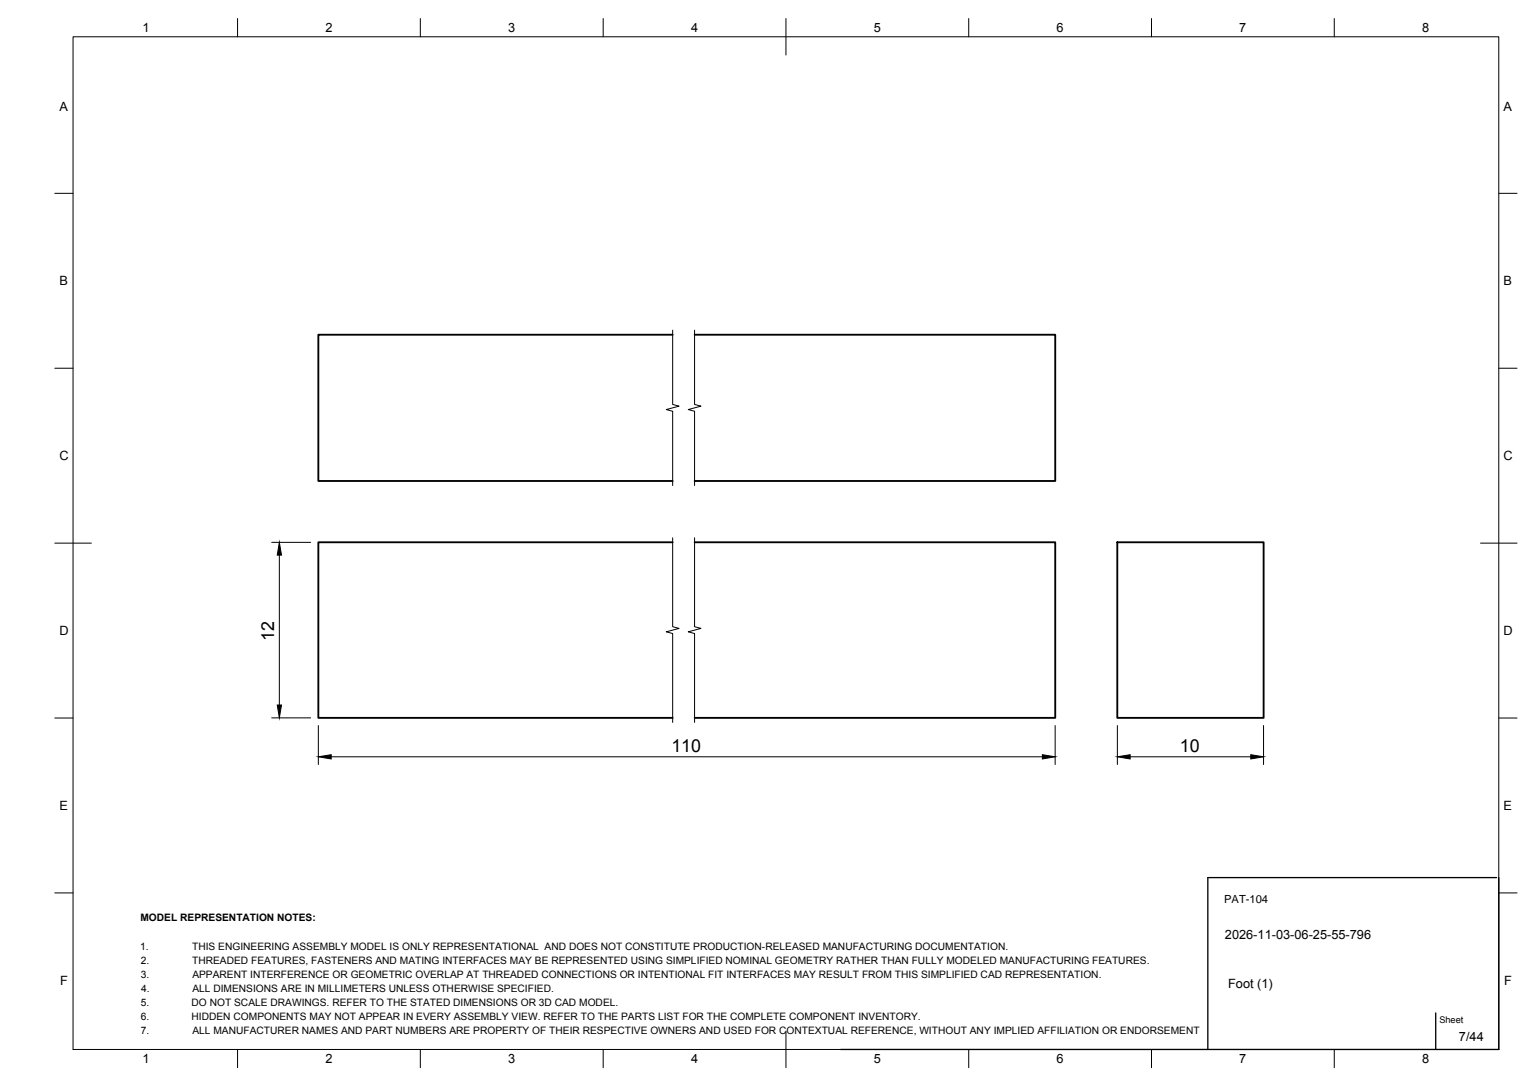
ISO-10303-21;
HEADER;
/* Generated by software containing ST-Developer
 * from STEP Tools, Inc. (www.steptools.com) 
 */

FILE_DESCRIPTION(
/* description */ ('Timing belt drive module 2 mm Pitch Timing 20T-40T'),

/* implementation_level */ '2;1');

FILE_NAME(
/* name */ 'Foot (1).step',
/* time_stamp */ '2026-10-28T03:25:12-07:00',
/* author */ (''),
/* organization */ (''),
/* preprocessor_version */ 'ST-DEVELOPER v20.2',
/* originating_system */ 'Autodesk Translation Framework v15.17.0.0',
/* authorisation */ '');

FILE_SCHEMA (('AUTOMOTIVE_DESIGN { 1 0 10303 214 3 1 1 }'));
ENDSEC;

DATA;
#10=MECHANICAL_DESIGN_GEOMETRIC_PRESENTATION_REPRESENTATION('',(#526),#17830);
#440=SHAPE_REPRESENTATION_RELATIONSHIP('SRR','None',#18010,#483);
#483=ADVANCED_BREP_SHAPE_REPRESENTATION('',(#584),#17785);
#526=STYLED_ITEM('',(#18331),#584);
#584=MANIFOLD_SOLID_BREP('Body1',#8983);
#797=PLANE('',#9585);
#798=PLANE('',#9586);
#799=PLANE('',#9587);
#800=PLANE('',#9588);
#801=PLANE('',#9589);
#802=PLANE('',#9590);
#998=FACE_OUTER_BOUND('',#1529,.T.);
#999=FACE_OUTER_BOUND('',#1530,.T.);
#1000=FACE_OUTER_BOUND('',#1531,.T.);
#1001=FACE_OUTER_BOUND('',#1532,.T.);
#1002=FACE_OUTER_BOUND('',#1533,.T.);
#1003=FACE_OUTER_BOUND('',#1534,.T.);
#1529=EDGE_LOOP('',(#5953,#5954,#5955,#5956));
#1530=EDGE_LOOP('',(#5957,#5958,#5959,#5960));
#1531=EDGE_LOOP('',(#5961,#5962,#5963,#5964));
#1532=EDGE_LOOP('',(#5965,#5966,#5967,#5968));
#1533=EDGE_LOOP('',(#5969,#5970,#5971,#5972));
#1534=EDGE_LOOP('',(#5973,#5974,#5975,#5976));
#2852=LINE('',#14067,#3330);
#2853=LINE('',#14069,#3331);
#2854=LINE('',#14071,#3332);
#2855=LINE('',#14072,#3333);
#2856=LINE('',#14075,#3334);
#2857=LINE('',#14077,#3335);
#2858=LINE('',#14078,#3336);
#2859=LINE('',#14081,#3337);
#2860=LINE('',#14083,#3338);
#2861=LINE('',#14084,#3339);
#2862=LINE('',#14086,#3340);
#2863=LINE('',#14087,#3341);
#3330=VECTOR('',#11011,1.);
#3331=VECTOR('',#11012,1.);
#3332=VECTOR('',#11013,1.);
#3333=VECTOR('',#11014,1.);
#3334=VECTOR('',#11017,1.);
#3335=VECTOR('',#11018,1.);
#3336=VECTOR('',#11019,1.);
#3337=VECTOR('',#11022,1.);
#3338=VECTOR('',#11023,1.);
#3339=VECTOR('',#11024,1.);
#3340=VECTOR('',#11027,1.);
#3341=VECTOR('',#11028,1.);
#3806=VERTEX_POINT('',#14065);
#3807=VERTEX_POINT('',#14066);
#3808=VERTEX_POINT('',#14068);
#3809=VERTEX_POINT('',#14070);
#3810=VERTEX_POINT('',#14074);
#3811=VERTEX_POINT('',#14076);
#3812=VERTEX_POINT('',#14080);
#3813=VERTEX_POINT('',#14082);
#4659=EDGE_CURVE('',#3806,#3807,#2852,.T.);
#4660=EDGE_CURVE('',#3807,#3808,#2853,.T.);
#4661=EDGE_CURVE('',#3809,#3808,#2854,.T.);
#4662=EDGE_CURVE('',#3806,#3809,#2855,.T.);
#4663=EDGE_CURVE('',#3810,#3806,#2856,.T.);
#4664=EDGE_CURVE('',#3811,#3809,#2857,.T.);
#4665=EDGE_CURVE('',#3810,#3811,#2858,.T.);
#4666=EDGE_CURVE('',#3812,#3810,#2859,.T.);
#4667=EDGE_CURVE('',#3813,#3811,#2860,.T.);
#4668=EDGE_CURVE('',#3812,#3813,#2861,.T.);
#4669=EDGE_CURVE('',#3807,#3812,#2862,.T.);
#4670=EDGE_CURVE('',#3808,#3813,#2863,.T.);
#5953=ORIENTED_EDGE('',*,*,#4659,.T.);
#5954=ORIENTED_EDGE('',*,*,#4660,.T.);
#5955=ORIENTED_EDGE('',*,*,#4661,.F.);
#5956=ORIENTED_EDGE('',*,*,#4662,.F.);
#5957=ORIENTED_EDGE('',*,*,#4663,.T.);
#5958=ORIENTED_EDGE('',*,*,#4662,.T.);
#5959=ORIENTED_EDGE('',*,*,#4664,.F.);
#5960=ORIENTED_EDGE('',*,*,#4665,.F.);
#5961=ORIENTED_EDGE('',*,*,#4666,.T.);
#5962=ORIENTED_EDGE('',*,*,#4665,.T.);
#5963=ORIENTED_EDGE('',*,*,#4667,.F.);
#5964=ORIENTED_EDGE('',*,*,#4668,.F.);
#5965=ORIENTED_EDGE('',*,*,#4669,.T.);
#5966=ORIENTED_EDGE('',*,*,#4668,.T.);
#5967=ORIENTED_EDGE('',*,*,#4670,.F.);
#5968=ORIENTED_EDGE('',*,*,#4660,.F.);
#5969=ORIENTED_EDGE('',*,*,#4670,.T.);
#5970=ORIENTED_EDGE('',*,*,#4667,.T.);
#5971=ORIENTED_EDGE('',*,*,#4664,.T.);
#5972=ORIENTED_EDGE('',*,*,#4661,.T.);
#5973=ORIENTED_EDGE('',*,*,#4669,.F.);
#5974=ORIENTED_EDGE('',*,*,#4659,.F.);
#5975=ORIENTED_EDGE('',*,*,#4663,.F.);
#5976=ORIENTED_EDGE('',*,*,#4666,.F.);
#8496=ADVANCED_FACE('',(#998),#797,.T.);
#8497=ADVANCED_FACE('',(#999),#798,.T.);
#8498=ADVANCED_FACE('',(#1000),#799,.T.);
#8499=ADVANCED_FACE('',(#1001),#800,.T.);
#8500=ADVANCED_FACE('',(#1002),#801,.T.);
#8501=ADVANCED_FACE('',(#1003),#802,.F.);
#8983=CLOSED_SHELL('',(#8496,#8497,#8498,#8499,#8500,#8501));
#9584=AXIS2_PLACEMENT_3D('',#14063,#11007,#11008);
#9585=AXIS2_PLACEMENT_3D('',#14064,#11009,#11010);
#9586=AXIS2_PLACEMENT_3D('',#14073,#11015,#11016);
#9587=AXIS2_PLACEMENT_3D('',#14079,#11020,#11021);
#9588=AXIS2_PLACEMENT_3D('',#14085,#11025,#11026);
#9589=AXIS2_PLACEMENT_3D('',#14088,#11029,#11030);
#9590=AXIS2_PLACEMENT_3D('',#14089,#11031,#11032);
#11007=DIRECTION('axis',(0.,0.,1.));
#11008=DIRECTION('refdir',(1.,0.,0.));
#11009=DIRECTION('center_axis',(0.,1.,0.));
#11010=DIRECTION('ref_axis',(-1.,0.,0.));
#11011=DIRECTION('',(-1.,0.,0.));
#11012=DIRECTION('',(0.,0.,1.));
#11013=DIRECTION('',(-1.,0.,0.));
#11014=DIRECTION('',(0.,0.,1.));
#11015=DIRECTION('center_axis',(1.,0.,0.));
#11016=DIRECTION('ref_axis',(0.,1.,0.));
#11017=DIRECTION('',(0.,1.,0.));
#11018=DIRECTION('',(0.,1.,0.));
#11019=DIRECTION('',(0.,0.,1.));
#11020=DIRECTION('center_axis',(0.,-1.,0.));
#11021=DIRECTION('ref_axis',(1.,0.,0.));
#11022=DIRECTION('',(1.,0.,0.));
#11023=DIRECTION('',(1.,0.,0.));
#11024=DIRECTION('',(0.,0.,1.));
#11025=DIRECTION('center_axis',(-1.,0.,0.));
#11026=DIRECTION('ref_axis',(0.,-1.,0.));
#11027=DIRECTION('',(0.,-1.,0.));
#11028=DIRECTION('',(0.,-1.,0.));
#11029=DIRECTION('center_axis',(0.,0.,1.));
#11030=DIRECTION('ref_axis',(1.,0.,0.));
#11031=DIRECTION('center_axis',(0.,0.,1.));
#11032=DIRECTION('ref_axis',(1.,0.,0.));
#14063=CARTESIAN_POINT('',(0.,0.,0.));
#14064=CARTESIAN_POINT('Origin',(12.,4.5,-2.4));
#14065=CARTESIAN_POINT('',(12.,4.5,-2.4));
#14066=CARTESIAN_POINT('',(11.,4.5,-2.4));
#14067=CARTESIAN_POINT('',(12.,4.5,-2.4));
#14068=CARTESIAN_POINT('',(11.,4.5,-1.2));
#14069=CARTESIAN_POINT('',(11.,4.5,-2.4));
#14070=CARTESIAN_POINT('',(12.,4.5,-1.2));
#14071=CARTESIAN_POINT('',(12.,4.5,-1.2));
#14072=CARTESIAN_POINT('',(12.,4.5,-2.4));
#14073=CARTESIAN_POINT('Origin',(12.,-6.5,-2.4));
#14074=CARTESIAN_POINT('',(12.,-6.5,-2.4));
#14075=CARTESIAN_POINT('',(12.,-6.5,-2.4));
#14076=CARTESIAN_POINT('',(12.,-6.5,-1.2));
#14077=CARTESIAN_POINT('',(12.,-6.5,-1.2));
#14078=CARTESIAN_POINT('',(12.,-6.5,-2.4));
#14079=CARTESIAN_POINT('Origin',(11.,-6.5,-2.4));
#14080=CARTESIAN_POINT('',(11.,-6.5,-2.4));
#14081=CARTESIAN_POINT('',(11.,-6.5,-2.4));
#14082=CARTESIAN_POINT('',(11.,-6.5,-1.2));
#14083=CARTESIAN_POINT('',(11.,-6.5,-1.2));
#14084=CARTESIAN_POINT('',(11.,-6.5,-2.4));
#14085=CARTESIAN_POINT('Origin',(11.,4.5,-2.4));
#14086=CARTESIAN_POINT('',(11.,4.5,-2.4));
#14087=CARTESIAN_POINT('',(11.,4.5,-1.2));
#14088=CARTESIAN_POINT('Origin',(11.5,-1.,-1.2));
#14089=CARTESIAN_POINT('Origin',(11.5,-1.,-2.4));
#17735=UNCERTAINTY_MEASURE_WITH_UNIT(LENGTH_MEASURE(0.001),#17831,
'DISTANCE_ACCURACY_VALUE',
'Maximum model space distance between geometric entities at asserted c
onnectivities');
#17780=UNCERTAINTY_MEASURE_WITH_UNIT(LENGTH_MEASURE(0.001),#17831,
'DISTANCE_ACCURACY_VALUE',
'Maximum model space distance between geometric entities at asserted c
onnectivities');
#17785=(
GEOMETRIC_REPRESENTATION_CONTEXT(3)
GLOBAL_UNCERTAINTY_ASSIGNED_CONTEXT((#17735))
GLOBAL_UNIT_ASSIGNED_CONTEXT((#17831,#17833,#17834))
REPRESENTATION_CONTEXT('','3D')
);
#17830=(
GEOMETRIC_REPRESENTATION_CONTEXT(3)
GLOBAL_UNCERTAINTY_ASSIGNED_CONTEXT((#17780))
GLOBAL_UNIT_ASSIGNED_CONTEXT((#17831,#17833,#17834))
REPRESENTATION_CONTEXT('','3D')
);
#17831=(
LENGTH_UNIT()
NAMED_UNIT(*)
SI_UNIT(.CENTI.,.METRE.)
);
#17833=(
NAMED_UNIT(*)
PLANE_ANGLE_UNIT()
SI_UNIT($,.RADIAN.)
);
#17834=(
NAMED_UNIT(*)
SI_UNIT($,.STERADIAN.)
SOLID_ANGLE_UNIT()
);
#17839=SHAPE_DEFINITION_REPRESENTATION(#17888,#18010);
#17888=PRODUCT_DEFINITION_SHAPE('',$,#18060);
#18010=SHAPE_REPRESENTATION('',(#9584),#17785);
#18055=PRODUCT_DEFINITION_CONTEXT('part definition',#18204,'design');
#18060=PRODUCT_DEFINITION('Foot (1)','Foot (1)',#18109,#18055);
#18109=PRODUCT_DEFINITION_FORMATION('',$,#18210);
#18204=APPLICATION_CONTEXT(
'Core Data for Automotive Mechanical Design Process');
#18205=PRODUCT_CONTEXT('part definition',#18204,'mechanical');
#18210=PRODUCT('Foot (1)','Foot (1)','Foot (1)',(#18205));
#18325=COLOUR_RGB('Off White',0.89,0.88,0.83);
#18326=FILL_AREA_STYLE_COLOUR('',#18325);
#18327=FILL_AREA_STYLE('',(#18326));
#18328=SURFACE_STYLE_FILL_AREA(#18327);
#18329=SURFACE_SIDE_STYLE('',(#18328));
#18330=SURFACE_STYLE_USAGE(.BOTH.,#18329);
#18331=PRESENTATION_STYLE_ASSIGNMENT((#18330));
ENDSEC;
END-ISO-10303-21;
